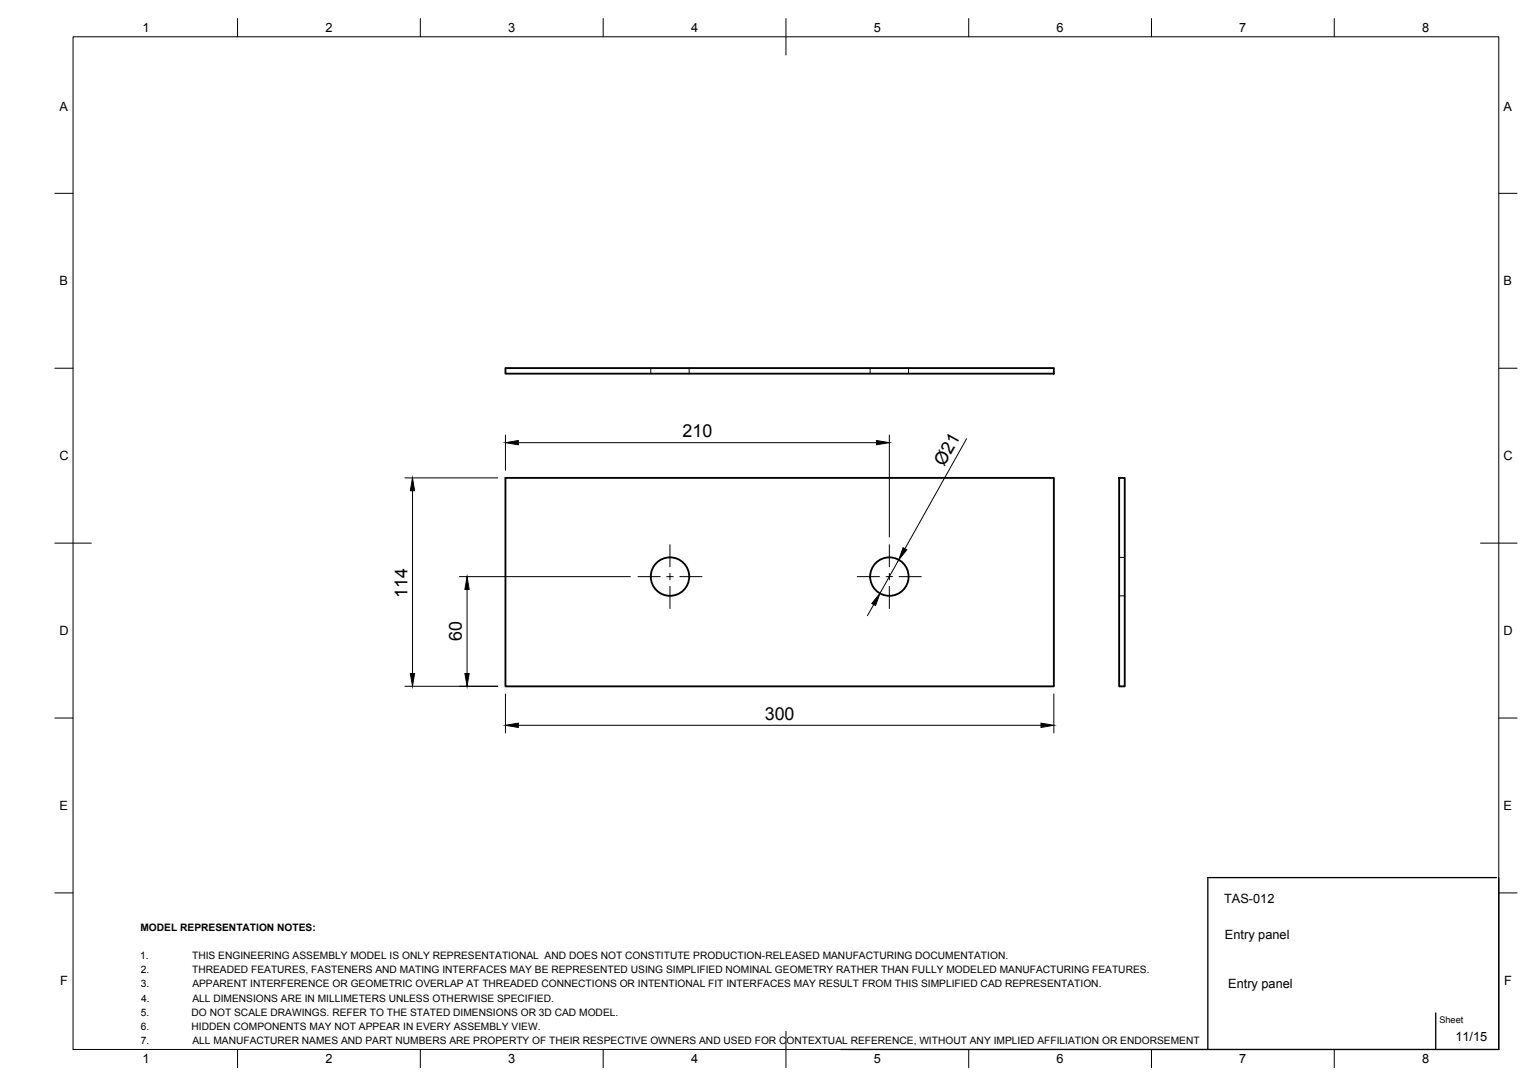
ISO-10303-21;
HEADER;
/* Generated by software containing ST-Developer
 * from STEP Tools, Inc. (www.steptools.com) 
 */

FILE_DESCRIPTION(
/* description */ (
'Independent welded steel electronics enclosure with removable sealed 
lid, internal mounting tray and two threaded cable entries. 300 x 220 
mm body. No ingress or electrical safety rating assigned.'),
/* implementation_level */ '2;1');

FILE_NAME(
/* name */ 'Entry panel.step',
/* time_stamp */ '2026-11-14T09:13:27-08:00',
/* author */ (''),
/* organization */ (''),
/* preprocessor_version */ 'ST-DEVELOPER v20.2',
/* originating_system */ 'Autodesk Translation Framework v15.17.0.0',
/* authorisation */ '');

FILE_SCHEMA (('AUTOMOTIVE_DESIGN { 1 0 10303 214 3 1 1 }'));
ENDSEC;

DATA;
#10=MECHANICAL_DESIGN_GEOMETRIC_PRESENTATION_REPRESENTATION('',(#967),#94412);
#937=SHAPE_REPRESENTATION_RELATIONSHIP('SRR','None',#94489,#952);
#952=ADVANCED_BREP_SHAPE_REPRESENTATION('',(#982),#94398);
#967=STYLED_ITEM('',(#94576),#982);
#982=MANIFOLD_SOLID_BREP('Body1',#8252);
#1004=FACE_BOUND('',#1535,.T.);
#1005=FACE_BOUND('',#1536,.T.);
#1006=FACE_BOUND('',#1539,.T.);
#1007=FACE_BOUND('',#1540,.T.);
#1064=PLANE('',#8460);
#1065=PLANE('',#8461);
#1066=PLANE('',#8462);
#1067=PLANE('',#8463);
#1068=PLANE('',#8464);
#1069=PLANE('',#8465);
#1168=FACE_OUTER_BOUND('',#1532,.T.);
#1169=FACE_OUTER_BOUND('',#1533,.T.);
#1170=FACE_OUTER_BOUND('',#1534,.T.);
#1171=FACE_OUTER_BOUND('',#1537,.T.);
#1172=FACE_OUTER_BOUND('',#1538,.T.);
#1173=FACE_OUTER_BOUND('',#1541,.T.);
#1174=FACE_OUTER_BOUND('',#1542,.T.);
#1175=FACE_OUTER_BOUND('',#1543,.T.);
#1532=EDGE_LOOP('',(#5142,#5143,#5144,#5145));
#1533=EDGE_LOOP('',(#5146,#5147,#5148,#5149));
#1534=EDGE_LOOP('',(#5150,#5151,#5152,#5153));
#1535=EDGE_LOOP('',(#5154));
#1536=EDGE_LOOP('',(#5155));
#1537=EDGE_LOOP('',(#5156,#5157,#5158,#5159));
#1538=EDGE_LOOP('',(#5160,#5161,#5162,#5163));
#1539=EDGE_LOOP('',(#5164));
#1540=EDGE_LOOP('',(#5165));
#1541=EDGE_LOOP('',(#5166,#5167,#5168,#5169));
#1542=EDGE_LOOP('',(#5170,#5171,#5172,#5173));
#1543=EDGE_LOOP('',(#5174,#5175,#5176,#5177));
#1948=LINE('',#10418,#2346);
#1949=LINE('',#10424,#2347);
#1950=LINE('',#10429,#2348);
#1951=LINE('',#10431,#2349);
#1952=LINE('',#10433,#2350);
#1953=LINE('',#10434,#2351);
#1954=LINE('',#10437,#2352);
#1955=LINE('',#10439,#2353);
#1956=LINE('',#10440,#2354);
#1957=LINE('',#10443,#2355);
#1958=LINE('',#10445,#2356);
#1959=LINE('',#10446,#2357);
#1960=LINE('',#10448,#2358);
#1961=LINE('',#10449,#2359);
#2346=VECTOR('',#9006,10.5);
#2347=VECTOR('',#9013,10.5);
#2348=VECTOR('',#9018,10.);
#2349=VECTOR('',#9019,10.);
#2350=VECTOR('',#9020,10.);
#2351=VECTOR('',#9021,10.);
#2352=VECTOR('',#9024,10.);
#2353=VECTOR('',#9025,10.);
#2354=VECTOR('',#9026,10.);
#2355=VECTOR('',#9029,10.);
#2356=VECTOR('',#9030,10.);
#2357=VECTOR('',#9031,10.);
#2358=VECTOR('',#9034,10.);
#2359=VECTOR('',#9035,10.);
#2736=CIRCLE('',#8455,10.5);
#2737=CIRCLE('',#8456,10.5);
#2738=CIRCLE('',#8458,10.5);
#2739=CIRCLE('',#8459,10.5);
#2862=VERTEX_POINT('',#10415);
#2863=VERTEX_POINT('',#10417);
#2864=VERTEX_POINT('',#10421);
#2865=VERTEX_POINT('',#10423);
#2866=VERTEX_POINT('',#10427);
#2867=VERTEX_POINT('',#10428);
#2868=VERTEX_POINT('',#10430);
#2869=VERTEX_POINT('',#10432);
#2870=VERTEX_POINT('',#10436);
#2871=VERTEX_POINT('',#10438);
#2872=VERTEX_POINT('',#10442);
#2873=VERTEX_POINT('',#10444);
#3836=EDGE_CURVE('',#2862,#2862,#2736,.T.);
#3837=EDGE_CURVE('',#2862,#2863,#1948,.T.);
#3838=EDGE_CURVE('',#2863,#2863,#2737,.T.);
#3839=EDGE_CURVE('',#2864,#2864,#2738,.T.);
#3840=EDGE_CURVE('',#2864,#2865,#1949,.T.);
#3841=EDGE_CURVE('',#2865,#2865,#2739,.T.);
#3842=EDGE_CURVE('',#2866,#2867,#1950,.T.);
#3843=EDGE_CURVE('',#2867,#2868,#1951,.T.);
#3844=EDGE_CURVE('',#2869,#2868,#1952,.T.);
#3845=EDGE_CURVE('',#2866,#2869,#1953,.T.);
#3846=EDGE_CURVE('',#2870,#2866,#1954,.T.);
#3847=EDGE_CURVE('',#2871,#2869,#1955,.T.);
#3848=EDGE_CURVE('',#2870,#2871,#1956,.T.);
#3849=EDGE_CURVE('',#2872,#2870,#1957,.T.);
#3850=EDGE_CURVE('',#2873,#2871,#1958,.T.);
#3851=EDGE_CURVE('',#2872,#2873,#1959,.T.);
#3852=EDGE_CURVE('',#2867,#2872,#1960,.T.);
#3853=EDGE_CURVE('',#2868,#2873,#1961,.T.);
#5142=ORIENTED_EDGE('',*,*,#3836,.F.);
#5143=ORIENTED_EDGE('',*,*,#3837,.T.);
#5144=ORIENTED_EDGE('',*,*,#3838,.F.);
#5145=ORIENTED_EDGE('',*,*,#3837,.F.);
#5146=ORIENTED_EDGE('',*,*,#3839,.F.);
#5147=ORIENTED_EDGE('',*,*,#3840,.T.);
#5148=ORIENTED_EDGE('',*,*,#3841,.F.);
#5149=ORIENTED_EDGE('',*,*,#3840,.F.);
#5150=ORIENTED_EDGE('',*,*,#3842,.T.);
#5151=ORIENTED_EDGE('',*,*,#3843,.T.);
#5152=ORIENTED_EDGE('',*,*,#3844,.F.);
#5153=ORIENTED_EDGE('',*,*,#3845,.F.);
#5154=ORIENTED_EDGE('',*,*,#3836,.T.);
#5155=ORIENTED_EDGE('',*,*,#3839,.T.);
#5156=ORIENTED_EDGE('',*,*,#3846,.T.);
#5157=ORIENTED_EDGE('',*,*,#3845,.T.);
#5158=ORIENTED_EDGE('',*,*,#3847,.F.);
#5159=ORIENTED_EDGE('',*,*,#3848,.F.);
#5160=ORIENTED_EDGE('',*,*,#3849,.T.);
#5161=ORIENTED_EDGE('',*,*,#3848,.T.);
#5162=ORIENTED_EDGE('',*,*,#3850,.F.);
#5163=ORIENTED_EDGE('',*,*,#3851,.F.);
#5164=ORIENTED_EDGE('',*,*,#3838,.T.);
#5165=ORIENTED_EDGE('',*,*,#3841,.T.);
#5166=ORIENTED_EDGE('',*,*,#3852,.T.);
#5167=ORIENTED_EDGE('',*,*,#3851,.T.);
#5168=ORIENTED_EDGE('',*,*,#3853,.F.);
#5169=ORIENTED_EDGE('',*,*,#3843,.F.);
#5170=ORIENTED_EDGE('',*,*,#3853,.T.);
#5171=ORIENTED_EDGE('',*,*,#3850,.T.);
#5172=ORIENTED_EDGE('',*,*,#3847,.T.);
#5173=ORIENTED_EDGE('',*,*,#3844,.T.);
#5174=ORIENTED_EDGE('',*,*,#3852,.F.);
#5175=ORIENTED_EDGE('',*,*,#3842,.F.);
#5176=ORIENTED_EDGE('',*,*,#3846,.F.);
#5177=ORIENTED_EDGE('',*,*,#3849,.F.);
#7662=CYLINDRICAL_SURFACE('',#8454,10.5);
#7663=CYLINDRICAL_SURFACE('',#8457,10.5);
#7905=ADVANCED_FACE('',(#1168),#7662,.F.);
#7906=ADVANCED_FACE('',(#1169),#7663,.F.);
#7907=ADVANCED_FACE('',(#1170,#1004,#1005),#1064,.T.);
#7908=ADVANCED_FACE('',(#1171),#1065,.T.);
#7909=ADVANCED_FACE('',(#1172,#1006,#1007),#1066,.T.);
#7910=ADVANCED_FACE('',(#1173),#1067,.T.);
#7911=ADVANCED_FACE('',(#1174),#1068,.T.);
#7912=ADVANCED_FACE('',(#1175),#1069,.F.);
#8252=CLOSED_SHELL('',(#7905,#7906,#7907,#7908,#7909,#7910,#7911,#7912));
#8453=AXIS2_PLACEMENT_3D('',#10413,#9000,#9001);
#8454=AXIS2_PLACEMENT_3D('',#10414,#9002,#9003);
#8455=AXIS2_PLACEMENT_3D('',#10416,#9004,#9005);
#8456=AXIS2_PLACEMENT_3D('',#10419,#9007,#9008);
#8457=AXIS2_PLACEMENT_3D('',#10420,#9009,#9010);
#8458=AXIS2_PLACEMENT_3D('',#10422,#9011,#9012);
#8459=AXIS2_PLACEMENT_3D('',#10425,#9014,#9015);
#8460=AXIS2_PLACEMENT_3D('',#10426,#9016,#9017);
#8461=AXIS2_PLACEMENT_3D('',#10435,#9022,#9023);
#8462=AXIS2_PLACEMENT_3D('',#10441,#9027,#9028);
#8463=AXIS2_PLACEMENT_3D('',#10447,#9032,#9033);
#8464=AXIS2_PLACEMENT_3D('',#10450,#9036,#9037);
#8465=AXIS2_PLACEMENT_3D('',#10451,#9038,#9039);
#9000=DIRECTION('axis',(0.,0.,1.));
#9001=DIRECTION('refdir',(1.,0.,0.));
#9002=DIRECTION('center_axis',(0.,-1.,0.));
#9003=DIRECTION('ref_axis',(0.,0.,1.));
#9004=DIRECTION('center_axis',(0.,-1.,0.));
#9005=DIRECTION('ref_axis',(0.,0.,1.));
#9006=DIRECTION('',(0.,-1.,0.));
#9007=DIRECTION('center_axis',(0.,1.,0.));
#9008=DIRECTION('ref_axis',(0.,0.,1.));
#9009=DIRECTION('center_axis',(0.,-1.,0.));
#9010=DIRECTION('ref_axis',(0.,0.,1.));
#9011=DIRECTION('center_axis',(0.,-1.,0.));
#9012=DIRECTION('ref_axis',(0.,0.,1.));
#9013=DIRECTION('',(0.,-1.,0.));
#9014=DIRECTION('center_axis',(0.,1.,0.));
#9015=DIRECTION('ref_axis',(0.,0.,1.));
#9016=DIRECTION('center_axis',(0.,1.,0.));
#9017=DIRECTION('ref_axis',(-1.,0.,0.));
#9018=DIRECTION('',(-1.,0.,0.));
#9019=DIRECTION('',(0.,0.,1.));
#9020=DIRECTION('',(-1.,0.,0.));
#9021=DIRECTION('',(0.,0.,1.));
#9022=DIRECTION('center_axis',(1.,0.,0.));
#9023=DIRECTION('ref_axis',(0.,1.,0.));
#9024=DIRECTION('',(0.,1.,0.));
#9025=DIRECTION('',(0.,1.,0.));
#9026=DIRECTION('',(0.,0.,1.));
#9027=DIRECTION('center_axis',(0.,-1.,0.));
#9028=DIRECTION('ref_axis',(1.,0.,0.));
#9029=DIRECTION('',(1.,0.,0.));
#9030=DIRECTION('',(1.,0.,0.));
#9031=DIRECTION('',(0.,0.,1.));
#9032=DIRECTION('center_axis',(-1.,0.,0.));
#9033=DIRECTION('ref_axis',(0.,-1.,0.));
#9034=DIRECTION('',(0.,-1.,0.));
#9035=DIRECTION('',(0.,-1.,0.));
#9036=DIRECTION('center_axis',(0.,0.,1.));
#9037=DIRECTION('ref_axis',(1.,0.,0.));
#9038=DIRECTION('center_axis',(0.,0.,1.));
#9039=DIRECTION('ref_axis',(1.,0.,0.));
#10413=CARTESIAN_POINT('',(0.,0.,0.));
#10414=CARTESIAN_POINT('Origin',(-60.,-2.77555756156289E-16,60.));
#10415=CARTESIAN_POINT('',(-60.,1.5,49.5));
#10416=CARTESIAN_POINT('Origin',(-60.,1.5,60.));
#10417=CARTESIAN_POINT('',(-60.,-1.5,49.5));
#10418=CARTESIAN_POINT('',(-60.,-2.77555756156289E-16,49.5));
#10419=CARTESIAN_POINT('Origin',(-60.,-1.5,60.));
#10420=CARTESIAN_POINT('Origin',(60.,-2.77555756156289E-16,60.));
#10421=CARTESIAN_POINT('',(60.,1.5,49.5));
#10422=CARTESIAN_POINT('Origin',(60.,1.5,60.));
#10423=CARTESIAN_POINT('',(60.,-1.5,49.5));
#10424=CARTESIAN_POINT('',(60.,-2.77555756156289E-16,49.5));
#10425=CARTESIAN_POINT('Origin',(60.,-1.5,60.));
#10426=CARTESIAN_POINT('Origin',(150.,1.5,0.));
#10427=CARTESIAN_POINT('',(150.,1.5,0.));
#10428=CARTESIAN_POINT('',(-150.,1.5,0.));
#10429=CARTESIAN_POINT('',(150.,1.5,0.));
#10430=CARTESIAN_POINT('',(-150.,1.5,114.));
#10431=CARTESIAN_POINT('',(-150.,1.5,0.));
#10432=CARTESIAN_POINT('',(150.,1.5,114.));
#10433=CARTESIAN_POINT('',(150.,1.5,114.));
#10434=CARTESIAN_POINT('',(150.,1.5,0.));
#10435=CARTESIAN_POINT('Origin',(150.,-1.5,0.));
#10436=CARTESIAN_POINT('',(150.,-1.5,0.));
#10437=CARTESIAN_POINT('',(150.,-1.5,0.));
#10438=CARTESIAN_POINT('',(150.,-1.5,114.));
#10439=CARTESIAN_POINT('',(150.,-1.5,114.));
#10440=CARTESIAN_POINT('',(150.,-1.5,0.));
#10441=CARTESIAN_POINT('Origin',(-150.,-1.5,0.));
#10442=CARTESIAN_POINT('',(-150.,-1.5,0.));
#10443=CARTESIAN_POINT('',(-150.,-1.5,0.));
#10444=CARTESIAN_POINT('',(-150.,-1.5,114.));
#10445=CARTESIAN_POINT('',(-150.,-1.5,114.));
#10446=CARTESIAN_POINT('',(-150.,-1.5,0.));
#10447=CARTESIAN_POINT('Origin',(-150.,1.5,0.));
#10448=CARTESIAN_POINT('',(-150.,1.5,0.));
#10449=CARTESIAN_POINT('',(-150.,1.5,114.));
#10450=CARTESIAN_POINT('Origin',(0.,0.,114.));
#10451=CARTESIAN_POINT('Origin',(0.,0.,0.));
#94380=UNCERTAINTY_MEASURE_WITH_UNIT(LENGTH_MEASURE(0.01),#94413,
'DISTANCE_ACCURACY_VALUE',
'Maximum model space distance between geometric entities at asserted c
onnectivities');
#94394=UNCERTAINTY_MEASURE_WITH_UNIT(LENGTH_MEASURE(0.01),#94413,
'DISTANCE_ACCURACY_VALUE',
'Maximum model space distance between geometric entities at asserted c
onnectivities');
#94398=(
GEOMETRIC_REPRESENTATION_CONTEXT(3)
GLOBAL_UNCERTAINTY_ASSIGNED_CONTEXT((#94380))
GLOBAL_UNIT_ASSIGNED_CONTEXT((#94413,#94415,#94416))
REPRESENTATION_CONTEXT('','3D')
);
#94412=(
GEOMETRIC_REPRESENTATION_CONTEXT(3)
GLOBAL_UNCERTAINTY_ASSIGNED_CONTEXT((#94394))
GLOBAL_UNIT_ASSIGNED_CONTEXT((#94413,#94415,#94416))
REPRESENTATION_CONTEXT('','3D')
);
#94413=(
LENGTH_UNIT()
NAMED_UNIT(*)
SI_UNIT(.MILLI.,.METRE.)
);
#94415=(
NAMED_UNIT(*)
PLANE_ANGLE_UNIT()
SI_UNIT($,.RADIAN.)
);
#94416=(
NAMED_UNIT(*)
SI_UNIT($,.STERADIAN.)
SOLID_ANGLE_UNIT()
);
#94420=SHAPE_DEFINITION_REPRESENTATION(#94437,#94489);
#94437=PRODUCT_DEFINITION_SHAPE('',$,#94507);
#94489=SHAPE_REPRESENTATION('',(#8453),#94398);
#94503=PRODUCT_DEFINITION_CONTEXT('part definition',#94556,'design');
#94507=PRODUCT_DEFINITION('Entry panel','Entry panel',#94524,#94503);
#94524=PRODUCT_DEFINITION_FORMATION('',$,#94561);
#94556=APPLICATION_CONTEXT(
'Core Data for Automotive Mechanical Design Process');
#94557=PRODUCT_CONTEXT('part definition',#94556,'mechanical');
#94561=PRODUCT('Entry panel','Entry panel',
'3 mm steel sheet; weld adjoining shell-panel edges continuously. Fabr
ication weld specification remains to be selected.',(#94557));
#94576=PRESENTATION_STYLE_ASSIGNMENT((#94583));
#94583=SURFACE_STYLE_USAGE(.BOTH.,#94590);
#94590=SURFACE_SIDE_STYLE('',(#94597));
#94597=SURFACE_STYLE_FILL_AREA(#94604);
#94604=FILL_AREA_STYLE('Opaque(23,69,131)',(#94611));
#94611=FILL_AREA_STYLE_COLOUR('Opaque(23,69,131)',#94618);
#94618=COLOUR_RGB('Opaque(23,69,131)',0.0901960784313725,0.270588235294118,
0.513725490196078);
ENDSEC;
END-ISO-10303-21;
